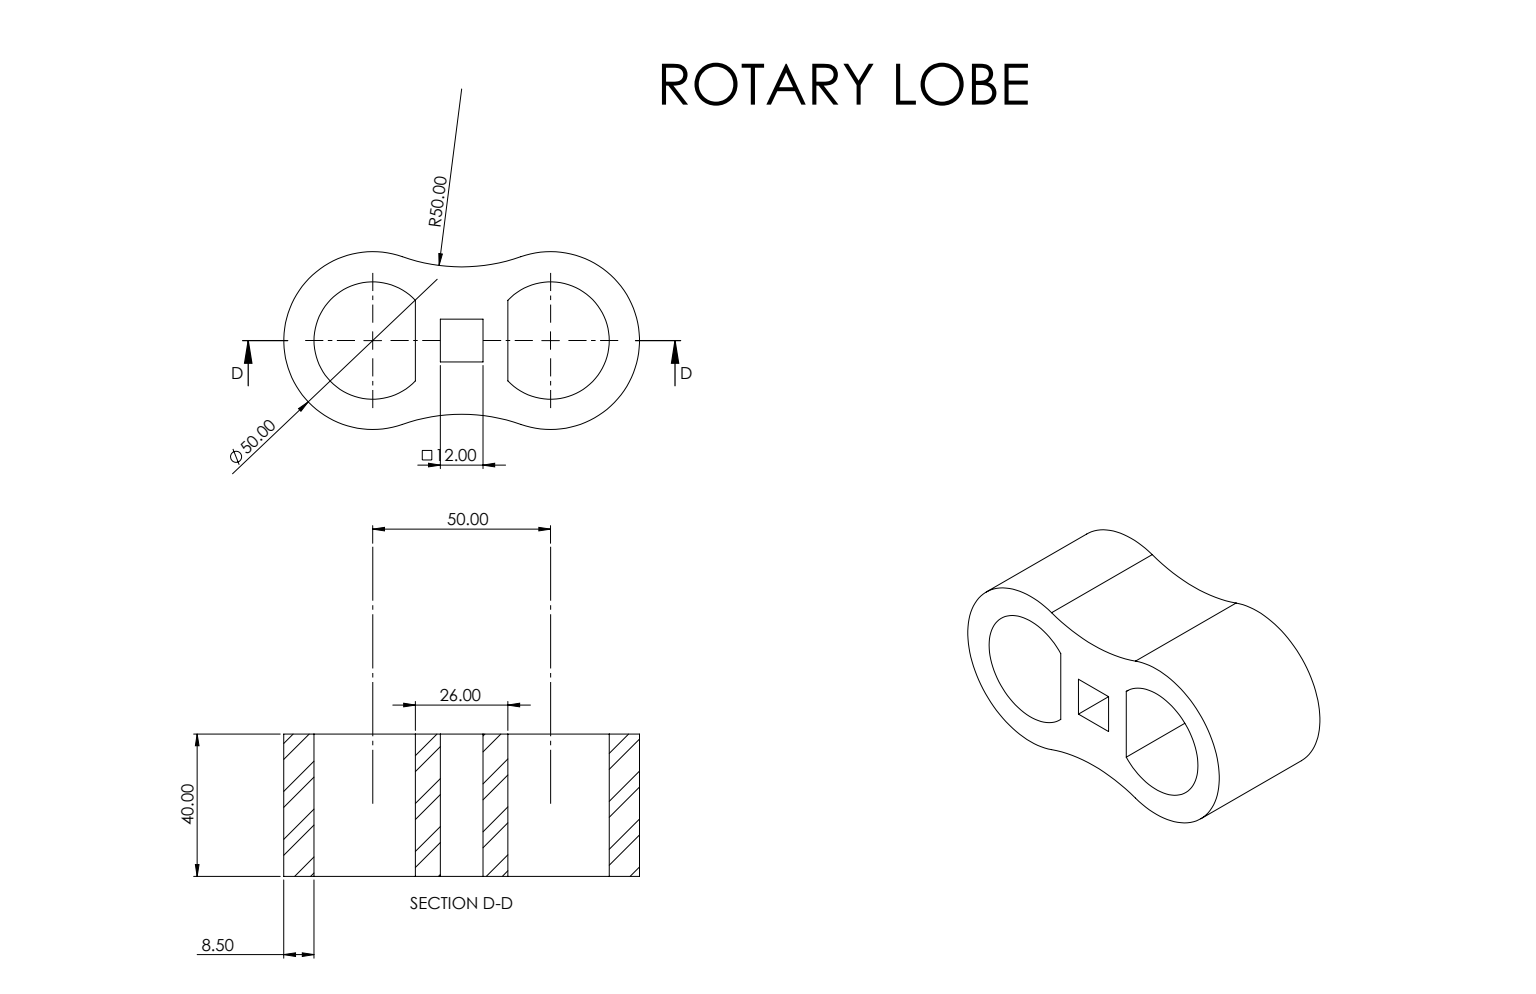
ISO-10303-21;
HEADER;
FILE_DESCRIPTION (('STEP AP214'),
    '1' );
FILE_NAME ('ROTARY LOBE.step',
    '2026-10-24T00:51:42',
    ( '' ),
    ( '' ),
    'SwSTEP 2.0',
    'SolidWorks 2025',
    '' );
FILE_SCHEMA (( 'AUTOMOTIVE_DESIGN' ));
ENDSEC;

DATA;
#53=DIRECTION ( 'NONE',  ( 0.000000000000000000, 0.000000000000000000, 1.000000000000000000 ) ) ;
#96=DIRECTION ( 'NONE',  ( -3.063596499322170048E-16, -0.000000000000000000, -1.000000000000000000 ) ) ;
#131=VERTEX_POINT ( 'NONE', #4797 ) ;
#159=VERTEX_POINT ( 'NONE', #1574 ) ;
#190=EDGE_CURVE ( 'NONE', #16687, #2945, #6029, .T. ) ;
#243=LINE ( 'NONE', #20894, #20346 ) ;
#257=ORIENTED_EDGE ( 'NONE', *, *, #16349, .T. ) ;
#306=PRODUCT_DEFINITION ( 'UNKNOWN', '', #18641, #21271 ) ;
#321=LINE ( 'NONE', #15778, #8511 ) ;
#407=VERTEX_POINT ( 'NONE', #7982 ) ;
#426=DIRECTION ( 'NONE',  ( -3.063596499322173499E-16, 0.000000000000000000, 1.000000000000000000 ) ) ;
#455=CYLINDRICAL_SURFACE ( 'NONE', #13115, 25.00000000000000000 ) ;
#462=DIRECTION ( 'NONE',  ( 0.000000000000000000, -0.000000000000000000, 1.000000000000000000 ) ) ;
#476=EDGE_CURVE ( 'NONE', #15630, #19286, #14390, .T. ) ;
#491=ORIENTED_EDGE ( 'NONE', *, *, #16782, .F. ) ;
#553=AXIS2_PLACEMENT_3D ( 'NONE', #10105, #20446, #6915 ) ;
#568=ORIENTED_EDGE ( 'NONE', *, *, #3531, .T. ) ;
#602=CARTESIAN_POINT ( 'NONE',  ( 25.00000000000000000, -20.00000000000000000, 6.487780019669002523E-15 ) ) ;
#631=DIRECTION ( 'NONE',  ( -0.000000000000000000, -1.000000000000000000, -0.000000000000000000 ) ) ;
#704=CARTESIAN_POINT ( 'NONE',  ( -5.999999999999998224, -20.00000000000000000, 5.999999999999999112 ) ) ;
#705=FACE_OUTER_BOUND ( 'NONE', #13898, .T. ) ;
#723=DIRECTION ( 'NONE',  ( 0.000000000000000000, 1.000000000000000000, -0.000000000000000000 ) ) ;
#779=CARTESIAN_POINT ( 'NONE',  ( -25.00000000000000000, -20.00000000000000000, 6.487780019669002523E-15 ) ) ;
#788=CARTESIAN_POINT ( 'NONE',  ( 12.99999999999999467, -20.00000000000000000, 11.32475165290614605 ) ) ;
#814=AXIS2_PLACEMENT_3D ( 'NONE', #20289, #11347, #21901 ) ;
#880=DIRECTION ( 'NONE',  ( 1.000000000000000000, 0.000000000000000000, 0.000000000000000000 ) ) ;
#893=EDGE_CURVE ( 'NONE', #11565, #12042, #19927, .T. ) ;
#919=AXIS2_PLACEMENT_3D ( 'NONE', #9251, #2386, #7658 ) ;
#965=ORIENTED_EDGE ( 'NONE', *, *, #15758, .T. ) ;
#974=VECTOR ( 'NONE', #96, 1000.000000000000000 ) ;
#989=CYLINDRICAL_SURFACE ( 'NONE', #17809, 16.49999999999998579 ) ;
#1008=DIRECTION ( 'NONE',  ( 0.000000000000000000, 1.000000000000000000, 0.000000000000000000 ) ) ;
#1069=EDGE_CURVE ( 'NONE', #407, #1418, #13674, .T. ) ;
#1071=FACE_OUTER_BOUND ( 'NONE', #3229, .T. ) ;
#1125=DIRECTION ( 'NONE',  ( 0.000000000000000000, 0.000000000000000000, -1.000000000000000000 ) ) ;
#1146=LINE ( 'NONE', #22009, #3920 ) ;
#1355=VECTOR ( 'NONE', #1852, 1000.000000000000000 ) ;
#1369=DIRECTION ( 'NONE',  ( -0.000000000000000000, -1.000000000000000000, -0.000000000000000000 ) ) ;
#1382=EDGE_CURVE ( 'NONE', #2473, #2421, #19105, .T. ) ;
#1401=CARTESIAN_POINT ( 'NONE',  ( -5.999999999999998224, 20.00000000000000000, 5.999999999999999112 ) ) ;
#1413=AXIS2_PLACEMENT_3D ( 'NONE', #7347, #12483, #462 ) ;
#1418=VERTEX_POINT ( 'NONE', #6415 ) ;
#1426=DIRECTION ( 'NONE',  ( 0.000000000000000000, 1.000000000000000000, 0.000000000000000000 ) ) ;
#1447=ORIENTED_EDGE ( 'NONE', *, *, #21089, .F. ) ;
#1523=DIRECTION ( 'NONE',  ( 0.000000000000000000, 0.000000000000000000, -1.000000000000000000 ) ) ;
#1574=CARTESIAN_POINT ( 'NONE',  ( -6.000000000000000000, -20.00000000000000000, -5.999999999999999112 ) ) ;
#1589=DIRECTION ( 'NONE',  ( 3.063596499322170048E-16, 0.000000000000000000, 1.000000000000000000 ) ) ;
#1621=DIRECTION ( 'NONE',  ( -0.000000000000000000, -1.000000000000000000, -0.000000000000000000 ) ) ;
#1648=CARTESIAN_POINT ( 'NONE',  ( 0.000000000000000000, 0.000000000000000000, 0.000000000000000000 ) ) ;
#1741=DIRECTION ( 'NONE',  ( 0.000000000000000000, 1.000000000000000000, 0.000000000000000000 ) ) ;
#1761=ORIENTED_EDGE ( 'NONE', *, *, #17671, .T. ) ;
#1773=DIRECTION ( 'NONE',  ( 0.000000000000000000, 0.000000000000000000, 1.000000000000000000 ) ) ;
#1790=AXIS2_PLACEMENT_3D ( 'NONE', #4562, #17989, #11540 ) ;
#1820=ORIENTED_EDGE ( 'NONE', *, *, #13645, .F. ) ;
#1849=CARTESIAN_POINT ( 'NONE',  ( -25.00000000000000000, 20.00000000000000000, 6.487780019669002523E-15 ) ) ;
#1852=DIRECTION ( 'NONE',  ( 1.445602896647339410E-16, 0.000000000000000000, 1.000000000000000000 ) ) ;
#1858=LINE ( 'NONE', #7117, #6849 ) ;
#1899=EDGE_LOOP ( 'NONE', ( #18124, #14504, #19988, #8484 ) ) ;
#1909=CARTESIAN_POINT ( 'NONE',  ( -25.00000000000000000, -20.00000000000000000, 6.487780019669002523E-15 ) ) ;
#1911=CARTESIAN_POINT ( 'NONE',  ( -16.66666666666665719, 20.00000000000000000, 23.57022603955159923 ) ) ;
#1936=ORIENTED_EDGE ( 'NONE', *, *, #18548, .F. ) ;
#2015=VERTEX_POINT ( 'NONE', #14566 ) ;
#2019=DIRECTION ( 'NONE',  ( 0.000000000000000000, 0.000000000000000000, 1.000000000000000000 ) ) ;
#2030=VERTEX_POINT ( 'NONE', #21576 ) ;
#2094=DIRECTION ( 'NONE',  ( 0.000000000000000000, 1.000000000000000000, -0.000000000000000000 ) ) ;
#2095=EDGE_LOOP ( 'NONE', ( #17339, #14563, #19602, #12820, #491, #11785, #13566, #22488, #22666 ) ) ;
#2119=ORIENTED_EDGE ( 'NONE', *, *, #11671, .T. ) ;
#2141=DIRECTION ( 'NONE',  ( -0.000000000000000000, -1.000000000000000000, -0.000000000000000000 ) ) ;
#2174=EDGE_LOOP ( 'NONE', ( #6678, #9947, #19944, #8878 ) ) ;
#2198=CIRCLE ( 'NONE', #18295, 25.00000000000000711 ) ;
#2229=AXIS2_PLACEMENT_3D ( 'NONE', #3378, #1426, #5315 ) ;
#2248=CARTESIAN_POINT ( 'NONE',  ( 25.00000000000000000, 20.00000000000000000, 6.487780019669002523E-15 ) ) ;
#2250=DIRECTION ( 'NONE',  ( 0.000000000000000000, 0.000000000000000000, 1.000000000000000000 ) ) ;
#2259=CARTESIAN_POINT ( 'NONE',  ( -5.999999999999998224, -20.00000000000000000, 5.999999999999999112 ) ) ;
#2279=CARTESIAN_POINT ( 'NONE',  ( 13.00000000000000178, 20.00000000000000000, -11.32475165290605901 ) ) ;
#2306=DIRECTION ( 'NONE',  ( -1.000000000000000000, 0.000000000000000000, 1.445602896647339410E-16 ) ) ;
#2312=ORIENTED_EDGE ( 'NONE', *, *, #5126, .F. ) ;
#2339=AXIS2_PLACEMENT_3D ( 'NONE', #13019, #1008, #21638 ) ;
#2378=LINE ( 'NONE', #18404, #11244 ) ;
#2386=DIRECTION ( 'NONE',  ( 0.000000000000000000, 1.000000000000000000, -0.000000000000000000 ) ) ;
#2421=VERTEX_POINT ( 'NONE', #8784 ) ;
#2433=EDGE_CURVE ( 'NONE', #17903, #10299, #3295, .T. ) ;
#2468=VECTOR ( 'NONE', #5542, 1000.000000000000000 ) ;
#2473=VERTEX_POINT ( 'NONE', #17595 ) ;
#2693=VERTEX_POINT ( 'NONE', #15154 ) ;
#2698=CARTESIAN_POINT ( 'NONE',  ( 12.99999999999999467, 20.00000000000000000, 11.32475165290614960 ) ) ;
#2712=DIRECTION ( 'NONE',  ( 0.000000000000000000, 1.000000000000000000, -0.000000000000000000 ) ) ;
#2728=FACE_OUTER_BOUND ( 'NONE', #6014, .T. ) ;
#2780=DIRECTION ( 'NONE',  ( -1.445602896647339410E-16, 0.000000000000000000, -1.000000000000000000 ) ) ;
#2792=LINE ( 'NONE', #4512, #19358 ) ;
#2818=DIRECTION ( 'NONE',  ( 0.000000000000000000, 1.000000000000000000, -0.000000000000000000 ) ) ;
#2827=ORIENTED_EDGE ( 'NONE', *, *, #14634, .T. ) ;
#2839=EDGE_CURVE ( 'NONE', #12042, #15630, #21166, .T. ) ;
#2900=( GEOMETRIC_REPRESENTATION_CONTEXT ( 3 ) GLOBAL_UNCERTAINTY_ASSIGNED_CONTEXT ( ( #11243 ) ) GLOBAL_UNIT_ASSIGNED_CONTEXT ( ( #17257, #8792, #12436 ) ) REPRESENTATION_CONTEXT ( 'NONE', 'WORKASPACE' ) );
#2913=DIRECTION ( 'NONE',  ( -0.000000000000000000, -1.000000000000000000, -0.000000000000000000 ) ) ;
#2945=VERTEX_POINT ( 'NONE', #19754 ) ;
#2970=CARTESIAN_POINT ( 'NONE',  ( -25.00000000000000000, 20.00000000000000000, -25.00000000000000000 ) ) ;
#2974=ORIENTED_EDGE ( 'NONE', *, *, #2433, .T. ) ;
#3037=ORIENTED_EDGE ( 'NONE', *, *, #16349, .F. ) ;
#3046=CARTESIAN_POINT ( 'NONE',  ( 16.66666666666669272, 20.00000000000000000, -23.57022603955159212 ) ) ;
#3095=LINE ( 'NONE', #14993, #11566 ) ;
#3102=AXIS2_PLACEMENT_3D ( 'NONE', #20493, #18423, #16830 ) ;
#3121=PLANE ( 'NONE',  #6042 ) ;
#3124=DIRECTION ( 'NONE',  ( 0.000000000000000000, 0.000000000000000000, 1.000000000000000000 ) ) ;
#3169=ORIENTED_EDGE ( 'NONE', *, *, #9920, .T. ) ;
#3200=ORIENTED_EDGE ( 'NONE', *, *, #6746, .F. ) ;
#3216=DIRECTION ( 'NONE',  ( 0.000000000000000000, 1.000000000000000000, 0.000000000000000000 ) ) ;
#3229=EDGE_LOOP ( 'NONE', ( #3200, #2312, #7838, #18951 ) ) ;
#3261=ORIENTED_EDGE ( 'NONE', *, *, #21083, .T. ) ;
#3262=AXIS2_PLACEMENT_3D ( 'NONE', #1849, #1621, #6664 ) ;
#3272=ADVANCED_FACE ( 'NONE', ( #15357 ), #10536, .T. ) ;
#3283=CIRCLE ( 'NONE', #18637, 25.00000000000000000 ) ;
#3295=LINE ( 'NONE', #19440, #19357 ) ;
#3327=LINE ( 'NONE', #6750, #20585 ) ;
#3378=CARTESIAN_POINT ( 'NONE',  ( -25.00000000000000000, 20.00000000000000000, 6.487780019669002523E-15 ) ) ;
#3430=SHAPE_REPRESENTATION ( 'ROTARY LOBE', ( #18273 ), #17150 ) ;
#3442=LINE ( 'NONE', #5489, #974 ) ;
#3484=CLOSED_SHELL ( 'NONE', ( #18863, #5857, #19734, #13310, #7530, #19685, #18289, #19085, #21947, #10343, #10632, #16278, #3272, #14244, #20666, #16635, #19070, #18858, #14622, #18536, #12603, #19793, #5819 ) ) ;
#3490=CARTESIAN_POINT ( 'NONE',  ( -12.99999999999999289, 20.00000000000000000, 11.32475165290611940 ) ) ;
#3521=VECTOR ( 'NONE', #15900, 1000.000000000000000 ) ;
#3531=EDGE_CURVE ( 'NONE', #2015, #20188, #12586, .T. ) ;
#3564=ORIENTED_EDGE ( 'NONE', *, *, #7437, .T. ) ;
#3585=ORIENTED_EDGE ( 'NONE', *, *, #21827, .F. ) ;
#3668=VECTOR ( 'NONE', #2141, 1000.000000000000000 ) ;
#3749=DIRECTION ( 'NONE',  ( 0.000000000000000000, 1.000000000000000000, 0.000000000000000000 ) ) ;
#3763=EDGE_CURVE ( 'NONE', #2693, #10299, #3327, .T. ) ;
#3765=CIRCLE ( 'NONE', #18773, 25.00000000000000000 ) ;
#3789=DIRECTION ( 'NONE',  ( 0.000000000000000000, 1.000000000000000000, 0.000000000000000000 ) ) ;
#3835=CARTESIAN_POINT ( 'NONE',  ( -16.66666666666665719, -20.00000000000000000, 23.57022603955159923 ) ) ;
#3837=AXIS2_PLACEMENT_3D ( 'NONE', #8979, #3838, #7382 ) ;
#3838=DIRECTION ( 'NONE',  ( 0.000000000000000000, 1.000000000000000000, 0.000000000000000000 ) ) ;
#3856=ORIENTED_EDGE ( 'NONE', *, *, #14469, .F. ) ;
#3860=EDGE_CURVE ( 'NONE', #17205, #20094, #321, .T. ) ;
#3864=CARTESIAN_POINT ( 'NONE',  ( -24.99999999999999645, 20.00000000000000000, 25.00000000000001421 ) ) ;
#3910=CARTESIAN_POINT ( 'NONE',  ( 5.999999999999998224, 20.00000000000000000, -5.999999999999999112 ) ) ;
#3920=VECTOR ( 'NONE', #22353, 1000.000000000000000 ) ;
#3955=VECTOR ( 'NONE', #12617, 1000.000000000000000 ) ;
#4012=DIRECTION ( 'NONE',  ( -0.000000000000000000, -1.000000000000000000, -0.000000000000000000 ) ) ;
#4017=AXIS2_PLACEMENT_3D ( 'NONE', #9577, #2712, #20128 ) ;
#4039=CARTESIAN_POINT ( 'NONE',  ( 25.00000000000000000, 20.00000000000000000, 6.487780019669002523E-15 ) ) ;
#4121=FACE_OUTER_BOUND ( 'NONE', #5496, .T. ) ;
#4164=CARTESIAN_POINT ( 'NONE',  ( -25.00000000000000000, 20.00000000000000000, -16.49999999999998934 ) ) ;
#4227=VECTOR ( 'NONE', #12091, 1000.000000000000000 ) ;
#4269=ORIENTED_EDGE ( 'NONE', *, *, #16752, .T. ) ;
#4276=DIRECTION ( 'NONE',  ( -0.000000000000000000, -1.000000000000000000, 0.000000000000000000 ) ) ;
#4325=AXIS2_PLACEMENT_3D ( 'NONE', #15578, #3789, #22601 ) ;
#4396=CARTESIAN_POINT ( 'NONE',  ( -25.00000000000000000, 20.00000000000000000, 6.487780019669002523E-15 ) ) ;
#4449=DIRECTION ( 'NONE',  ( 0.000000000000000000, 1.000000000000000000, 0.000000000000000000 ) ) ;
#4454=ORIENTED_EDGE ( 'NONE', *, *, #893, .T. ) ;
#4512=CARTESIAN_POINT ( 'NONE',  ( -16.66666666666665719, 20.00000000000000000, 23.57022603955159923 ) ) ;
#4516=EDGE_CURVE ( 'NONE', #5200, #16687, #22138, .T. ) ;
#4517=ORIENTED_EDGE ( 'NONE', *, *, #11352, .F. ) ;
#4562=CARTESIAN_POINT ( 'NONE',  ( -25.00000000000000000, 20.00000000000000000, 6.487780019669002523E-15 ) ) ;
#4571=DIRECTION ( 'NONE',  ( -0.000000000000000000, -1.000000000000000000, -0.000000000000000000 ) ) ;
#4602=CARTESIAN_POINT ( 'NONE',  ( 1.734723475976807094E-14, -20.00000000000000000, 70.71067811865476926 ) ) ;
#4624=DIRECTION ( 'NONE',  ( -0.000000000000000000, -1.000000000000000000, -0.000000000000000000 ) ) ;
#4657=CARTESIAN_POINT ( 'NONE',  ( 5.999999999999998224, -20.00000000000000000, -5.999999999999999112 ) ) ;
#4662=CARTESIAN_POINT ( 'NONE',  ( 1.734723475976807094E-14, -20.00000000000000000, 70.71067811865476926 ) ) ;
#4702=VECTOR ( 'NONE', #426, 1000.000000000000000 ) ;
#4754=CARTESIAN_POINT ( 'NONE',  ( -6.000000000000000000, 20.00000000000000000, -5.999999999999999112 ) ) ;
#4770=AXIS2_PLACEMENT_3D ( 'NONE', #15418, #4571, #1125 ) ;
#4796=ORIENTED_EDGE ( 'NONE', *, *, #20868, .F. ) ;
#4797=CARTESIAN_POINT ( 'NONE',  ( 25.00000000000000000, -20.00000000000000000, -24.99999999999999289 ) ) ;
#4835=CARTESIAN_POINT ( 'NONE',  ( -25.00000000000000000, 20.00000000000000000, 6.487780019669002523E-15 ) ) ;
#4867=LINE ( 'NONE', #13888, #5896 ) ;
#4885=ORIENTED_EDGE ( 'NONE', *, *, #9185, .T. ) ;
#4921=DIRECTION ( 'NONE',  ( -1.000000000000000000, 0.000000000000000000, 3.063596499322170048E-16 ) ) ;
#4932=CARTESIAN_POINT ( 'NONE',  ( -24.99999999999999645, 20.00000000000000000, 16.50000000000000355 ) ) ;
#4958=CARTESIAN_POINT ( 'NONE',  ( 25.00000000000000000, 20.00000000000000000, 6.487780019669002523E-15 ) ) ;
#4980=CARTESIAN_POINT ( 'NONE',  ( -25.00000000000000000, -20.00000000000000000, 6.487780019669002523E-15 ) ) ;
#4983=CIRCLE ( 'NONE', #6815, 16.49999999999999645 ) ;
#5034=LINE ( 'NONE', #6406, #18207 ) ;
#5063=SHAPE_DEFINITION_REPRESENTATION ( #14396, #3430 ) ;
#5089=CARTESIAN_POINT ( 'NONE',  ( -25.00000000000000000, 20.00000000000000000, 6.487780019669002523E-15 ) ) ;
#5126=EDGE_CURVE ( 'NONE', #11767, #20985, #19755, .T. ) ;
#5128=DIRECTION ( 'NONE',  ( -3.063596499322170048E-16, -0.000000000000000000, -1.000000000000000000 ) ) ;
#5158=FACE_OUTER_BOUND ( 'NONE', #5317, .T. ) ;
#5200=VERTEX_POINT ( 'NONE', #4164 ) ;
#5251=CIRCLE ( 'NONE', #3837, 25.00000000000000000 ) ;
#5272=LINE ( 'NONE', #11789, #21724 ) ;
#5281=AXIS2_PLACEMENT_3D ( 'NONE', #7089, #3216, #15441 ) ;
#5315=DIRECTION ( 'NONE',  ( 0.000000000000000000, 0.000000000000000000, 1.000000000000000000 ) ) ;
#5317=EDGE_LOOP ( 'NONE', ( #10062, #14422, #7754, #15956 ) ) ;
#5371=CARTESIAN_POINT ( 'NONE',  ( -25.00000000000000000, 20.00000000000000000, 6.487780019669002523E-15 ) ) ;
#5418=ORIENTED_EDGE ( 'NONE', *, *, #3860, .F. ) ;
#5489=CARTESIAN_POINT ( 'NONE',  ( -13.00000000000000178, 20.00000000000000000, -11.32475165290611407 ) ) ;
#5492=CARTESIAN_POINT ( 'NONE',  ( -5.999999999999998224, 20.00000000000000000, 5.999999999999999112 ) ) ;
#5496=EDGE_LOOP ( 'NONE', ( #9868, #6218, #10357, #19825 ) ) ;
#5516=DIRECTION ( 'NONE',  ( -0.000000000000000000, -1.000000000000000000, -0.000000000000000000 ) ) ;
#5542=DIRECTION ( 'NONE',  ( -0.000000000000000000, -1.000000000000000000, -0.000000000000000000 ) ) ;
#5613=DIRECTION ( 'NONE',  ( -0.000000000000000000, -1.000000000000000000, -0.000000000000000000 ) ) ;
#5628=VECTOR ( 'NONE', #880, 1000.000000000000000 ) ;
#5630=VERTEX_POINT ( 'NONE', #11344 ) ;
#5653=CARTESIAN_POINT ( 'NONE',  ( 25.00000000000000355, 20.00000000000000000, 16.49999999999999289 ) ) ;
#5715=ORIENTED_EDGE ( 'NONE', *, *, #17671, .F. ) ;
#5755=( NAMED_UNIT ( * ) SI_UNIT ( $, .STERADIAN. ) SOLID_ANGLE_UNIT ( ) );
#5768=DIRECTION ( 'NONE',  ( 0.000000000000000000, 0.000000000000000000, 1.000000000000000000 ) ) ;
#5819=ADVANCED_FACE ( 'NONE', ( #5158 ), #6983, .T. ) ;
#5829=PRODUCT ( 'ROTARY LOBE', 'ROTARY LOBE', '', ( #10300 ) ) ;
#5840=DIRECTION ( 'NONE',  ( 1.000000000000000000, -0.000000000000000000, 3.063596499322173499E-16 ) ) ;
#5857=ADVANCED_FACE ( 'NONE', ( #12023 ), #15673, .F. ) ;
#5892=DIRECTION ( 'NONE',  ( 1.000000000000000000, 0.000000000000000000, -0.000000000000000000 ) ) ;
#5896=VECTOR ( 'NONE', #19298, 1000.000000000000000 ) ;
#5949=EDGE_CURVE ( 'NONE', #11275, #11481, #9145, .T. ) ;
#5975=ORIENTED_EDGE ( 'NONE', *, *, #12491, .F. ) ;
#5999=LINE ( 'NONE', #7490, #7179 ) ;
#6014=EDGE_LOOP ( 'NONE', ( #13694, #2827, #8705, #18362 ) ) ;
#6028=EDGE_CURVE ( 'NONE', #2421, #11565, #13451, .T. ) ;
#6029=CIRCLE ( 'NONE', #18836, 16.49999999999999645 ) ;
#6030=DIRECTION ( 'NONE',  ( 0.000000000000000000, 1.000000000000000000, 0.000000000000000000 ) ) ;
#6041=DIRECTION ( 'NONE',  ( 1.445602896647339410E-16, 0.000000000000000000, 1.000000000000000000 ) ) ;
#6042=AXIS2_PLACEMENT_3D ( 'NONE', #1401, #8059, #15362 ) ;
#6048=LINE ( 'NONE', #13015, #15559 ) ;
#6117=DIRECTION ( 'NONE',  ( -0.000000000000000000, -1.000000000000000000, -0.000000000000000000 ) ) ;
#6161=LINE ( 'NONE', #2259, #5628 ) ;
#6218=ORIENTED_EDGE ( 'NONE', *, *, #9082, .F. ) ;
#6330=LINE ( 'NONE', #13289, #10426 ) ;
#6337=EDGE_CURVE ( 'NONE', #17762, #15630, #2792, .T. ) ;
#6406=CARTESIAN_POINT ( 'NONE',  ( -25.00000000000000000, 20.00000000000000000, -25.00000000000000000 ) ) ;
#6415=CARTESIAN_POINT ( 'NONE',  ( 13.00000000000000178, 20.00000000000000000, -11.32475165290605723 ) ) ;
#6436=CARTESIAN_POINT ( 'NONE',  ( -25.00000000000000000, 20.00000000000000000, -16.49999999999998934 ) ) ;
#6458=FACE_OUTER_BOUND ( 'NONE', #7366, .T. ) ;
#6459=FACE_OUTER_BOUND ( 'NONE', #9454, .T. ) ;
#6555=FACE_OUTER_BOUND ( 'NONE', #18849, .T. ) ;
#6598=DIRECTION ( 'NONE',  ( -0.000000000000000000, -1.000000000000000000, 0.000000000000000000 ) ) ;
#6649=DIRECTION ( 'NONE',  ( -0.000000000000000000, -1.000000000000000000, -0.000000000000000000 ) ) ;
#6664=DIRECTION ( 'NONE',  ( 0.000000000000000000, 0.000000000000000000, -1.000000000000000000 ) ) ;
#6675=CYLINDRICAL_SURFACE ( 'NONE', #20729, 25.00000000000000000 ) ;
#6678=ORIENTED_EDGE ( 'NONE', *, *, #15968, .F. ) ;
#6700=EDGE_LOOP ( 'NONE', ( #9292, #1761, #17911, #7155 ) ) ;
#6720=DIRECTION ( 'NONE',  ( -0.000000000000000000, -1.000000000000000000, -0.000000000000000000 ) ) ;
#6746=EDGE_CURVE ( 'NONE', #20985, #9978, #6161, .T. ) ;
#6750=CARTESIAN_POINT ( 'NONE',  ( -13.00000000000000178, 20.00000000000000000, -11.32475165290611407 ) ) ;
#6763=DIRECTION ( 'NONE',  ( 0.000000000000000000, 0.000000000000000000, -1.000000000000000000 ) ) ;
#6815=AXIS2_PLACEMENT_3D ( 'NONE', #4396, #16528, #5768 ) ;
#6849=VECTOR ( 'NONE', #14663, 1000.000000000000000 ) ;
#6866=CIRCLE ( 'NONE', #4325, 25.00000000000000000 ) ;
#6903=CARTESIAN_POINT ( 'NONE',  ( -25.00000000000000000, -20.00000000000000000, 6.487780019669002523E-15 ) ) ;
#6915=DIRECTION ( 'NONE',  ( 0.000000000000000000, 0.000000000000000000, -1.000000000000000000 ) ) ;
#6983=PLANE ( 'NONE',  #11266 ) ;
#6988=FACE_BOUND ( 'NONE', #8101, .T. ) ;
#6994=DIRECTION ( 'NONE',  ( 0.000000000000000000, 0.000000000000000000, 1.000000000000000000 ) ) ;
#7089=CARTESIAN_POINT ( 'NONE',  ( 12.50000000000000888, -20.00000000000000000, -35.35533905932738463 ) ) ;
#7117=CARTESIAN_POINT ( 'NONE',  ( -24.99999999999999645, 20.00000000000000000, 16.50000000000000355 ) ) ;
#7155=ORIENTED_EDGE ( 'NONE', *, *, #5949, .T. ) ;
#7176=AXIS2_PLACEMENT_3D ( 'NONE', #11793, #8145, #14999 ) ;
#7179=VECTOR ( 'NONE', #6117, 1000.000000000000000 ) ;
#7291=VERTEX_POINT ( 'NONE', #2698 ) ;
#7324=VERTEX_POINT ( 'NONE', #14931 ) ;
#7347=CARTESIAN_POINT ( 'NONE',  ( 12.50000000000000888, 20.00000000000000000, -35.35533905932738463 ) ) ;
#7360=( LENGTH_UNIT ( ) NAMED_UNIT ( * ) SI_UNIT ( .MILLI., .METRE. ) );
#7366=EDGE_LOOP ( 'NONE', ( #1936, #14220, #9943, #22495 ) ) ;
#7369=ORIENTED_EDGE ( 'NONE', *, *, #18515, .F. ) ;
#7382=DIRECTION ( 'NONE',  ( 0.000000000000000000, 0.000000000000000000, 1.000000000000000000 ) ) ;
#7405=CYLINDRICAL_SURFACE ( 'NONE', #10592, 16.49999999999998579 ) ;
#7412=ORIENTED_EDGE ( 'NONE', *, *, #1069, .T. ) ;
#7437=EDGE_CURVE ( 'NONE', #16688, #12891, #8914, .T. ) ;
#7490=CARTESIAN_POINT ( 'NONE',  ( -12.99999999999999467, 20.00000000000000000, 11.32475165290612296 ) ) ;
#7530=ADVANCED_FACE ( 'NONE', ( #18165 ), #11164, .T. ) ;
#7549=EDGE_LOOP ( 'NONE', ( #3169, #12624, #4885, #2974 ) ) ;
#7601=AXIS2_PLACEMENT_3D ( 'NONE', #18464, #10083, #2780 ) ;
#7608=DIRECTION ( 'NONE',  ( 0.000000000000000000, 0.000000000000000000, 1.000000000000000000 ) ) ;
#7658=DIRECTION ( 'NONE',  ( 0.000000000000000000, 0.000000000000000000, -1.000000000000000000 ) ) ;
#7671=ORIENTED_EDGE ( 'NONE', *, *, #18661, .F. ) ;
#7687=FACE_BOUND ( 'NONE', #1899, .T. ) ;
#7698=ORIENTED_EDGE ( 'NONE', *, *, #7997, .T. ) ;
#7749=EDGE_CURVE ( 'NONE', #16771, #7803, #12104, .T. ) ;
#7754=ORIENTED_EDGE ( 'NONE', *, *, #15877, .T. ) ;
#7775=EDGE_CURVE ( 'NONE', #2030, #9978, #4867, .T. ) ;
#7803=VERTEX_POINT ( 'NONE', #3490 ) ;
#7838=ORIENTED_EDGE ( 'NONE', *, *, #13992, .T. ) ;
#7872=AXIS2_PLACEMENT_3D ( 'NONE', #4662, #6598, #13562 ) ;
#7938=ORIENTED_EDGE ( 'NONE', *, *, #476, .T. ) ;
#7953=EDGE_LOOP ( 'NONE', ( #1447, #12865, #17410, #2119 ) ) ;
#7982=CARTESIAN_POINT ( 'NONE',  ( 25.00000000000000000, 20.00000000000000000, -16.49999999999997868 ) ) ;
#7985=ORIENTED_EDGE ( 'NONE', *, *, #18946, .T. ) ;
#7990=CIRCLE ( 'NONE', #18236, 16.49999999999999645 ) ;
#7997=EDGE_CURVE ( 'NONE', #17762, #10374, #22371, .T. ) ;
#8000=FACE_OUTER_BOUND ( 'NONE', #21573, .T. ) ;
#8059=DIRECTION ( 'NONE',  ( 0.000000000000000000, 0.000000000000000000, -1.000000000000000000 ) ) ;
#8101=EDGE_LOOP ( 'NONE', ( #965, #15077, #19109, #13023 ) ) ;
#8105=FACE_OUTER_BOUND ( 'NONE', #10982, .T. ) ;
#8145=DIRECTION ( 'NONE',  ( 0.000000000000000000, 1.000000000000000000, 0.000000000000000000 ) ) ;
#8174=DIRECTION ( 'NONE',  ( -0.000000000000000000, -1.000000000000000000, -0.000000000000000000 ) ) ;
#8175=DIRECTION ( 'NONE',  ( 0.000000000000000000, 1.000000000000000000, 0.000000000000000000 ) ) ;
#8222=AXIS2_PLACEMENT_3D ( 'NONE', #9939, #13699, #17038 ) ;
#8233=EDGE_LOOP ( 'NONE', ( #17203, #16857, #11709, #19544 ) ) ;
#8344=AXIS2_PLACEMENT_3D ( 'NONE', #20252, #6720, #11536 ) ;
#8364=VERTEX_POINT ( 'NONE', #14301 ) ;
#8369=ORIENTED_EDGE ( 'NONE', *, *, #17783, .T. ) ;
#8371=CARTESIAN_POINT ( 'NONE',  ( 1.734723475976807094E-14, 20.00000000000000000, -70.71067811865476926 ) ) ;
#8382=CYLINDRICAL_SURFACE ( 'NONE', #17110, 16.49999999999999645 ) ;
#8384=VERTEX_POINT ( 'NONE', #10994 ) ;
#8396=FACE_OUTER_BOUND ( 'NONE', #7953, .T. ) ;
#8484=ORIENTED_EDGE ( 'NONE', *, *, #17041, .F. ) ;
#8507=CYLINDRICAL_SURFACE ( 'NONE', #553, 50.00000000000001421 ) ;
#8511=VECTOR ( 'NONE', #21521, 1000.000000000000000 ) ;
#8522=ORIENTED_EDGE ( 'NONE', *, *, #11352, .T. ) ;
#8594=ORIENTED_EDGE ( 'NONE', *, *, #13992, .F. ) ;
#8623=VECTOR ( 'NONE', #10210, 1000.000000000000000 ) ;
#8698=AXIS2_PLACEMENT_3D ( 'NONE', #5371, #21522, #12791 ) ;
#8705=ORIENTED_EDGE ( 'NONE', *, *, #13539, .T. ) ;
#8772=CARTESIAN_POINT ( 'NONE',  ( 25.00000000000000000, -20.00000000000000000, 6.487780019669002523E-15 ) ) ;
#8784=CARTESIAN_POINT ( 'NONE',  ( -16.66666666666666785, -20.00000000000000000, -23.57022603955158502 ) ) ;
#8792=( NAMED_UNIT ( * ) PLANE_ANGLE_UNIT ( ) SI_UNIT ( $, .RADIAN. ) );
#8850=SHAPE_REPRESENTATION_RELATIONSHIP ( 'NONE' , 'NONE' ,  #3430, #14250 ) ;
#8878=ORIENTED_EDGE ( 'NONE', *, *, #13645, .T. ) ;
#8914=CIRCLE ( 'NONE', #2339, 25.00000000000000711 ) ;
#8943=DIRECTION ( 'NONE',  ( 0.000000000000000000, 0.000000000000000000, -1.000000000000000000 ) ) ;
#8973=VERTEX_POINT ( 'NONE', #10790 ) ;
#8979=CARTESIAN_POINT ( 'NONE',  ( 25.00000000000000000, 20.00000000000000000, 6.487780019669002523E-15 ) ) ;
#8988=VERTEX_POINT ( 'NONE', #17912 ) ;
#9082=EDGE_CURVE ( 'NONE', #1418, #11275, #11600, .T. ) ;
#9128=DIRECTION ( 'NONE',  ( 0.000000000000000000, 0.000000000000000000, -1.000000000000000000 ) ) ;
#9145=LINE ( 'NONE', #16116, #4702 ) ;
#9185=EDGE_CURVE ( 'NONE', #2945, #17903, #20404, .T. ) ;
#9213=EDGE_CURVE ( 'NONE', #159, #20985, #10089, .T. ) ;
#9251=CARTESIAN_POINT ( 'NONE',  ( 25.00000000000000000, -20.00000000000000000, 6.487780019669002523E-15 ) ) ;
#9292=ORIENTED_EDGE ( 'NONE', *, *, #14469, .T. ) ;
#9357=CARTESIAN_POINT ( 'NONE',  ( 25.00000000000000000, 20.00000000000000000, 6.487780019669002523E-15 ) ) ;
#9360=DIRECTION ( 'NONE',  ( -0.000000000000000000, -1.000000000000000000, -0.000000000000000000 ) ) ;
#9368=ORIENTED_EDGE ( 'NONE', *, *, #16106, .F. ) ;
#9437=ORIENTED_EDGE ( 'NONE', *, *, #4516, .F. ) ;
#9454=EDGE_LOOP ( 'NONE', ( #12266, #22168, #5975, #14521 ) ) ;
#9487=MECHANICAL_DESIGN_GEOMETRIC_PRESENTATION_REPRESENTATION('',(#9844),#2900);
#9577=CARTESIAN_POINT ( 'NONE',  ( 25.00000000000000000, 20.00000000000000000, 6.487780019669002523E-15 ) ) ;
#9761=DIRECTION ( 'NONE',  ( 0.000000000000000000, 0.000000000000000000, -1.000000000000000000 ) ) ;
#9762=DIRECTION ( 'NONE',  ( 0.000000000000000000, 0.000000000000000000, -1.000000000000000000 ) ) ;
#9774=CARTESIAN_POINT ( 'NONE',  ( -25.00000000000000000, -20.00000000000000000, 6.487780019669002523E-15 ) ) ;
#9835=CYLINDRICAL_SURFACE ( 'NONE', #4770, 50.00000000000000000 ) ;
#9844=STYLED_ITEM('',(#22720),#17752);
#9850=ORIENTED_EDGE ( 'NONE', *, *, #9185, .F. ) ;
#9868=ORIENTED_EDGE ( 'NONE', *, *, #5949, .F. ) ;
#9884=DIRECTION ( 'NONE',  ( 0.000000000000000000, 1.000000000000000000, 0.000000000000000000 ) ) ;
#9920=EDGE_CURVE ( 'NONE', #10299, #16687, #7990, .T. ) ;
#9939=CARTESIAN_POINT ( 'NONE',  ( 1.734723475976807094E-14, 20.00000000000000000, 70.71067811865476926 ) ) ;
#9943=ORIENTED_EDGE ( 'NONE', *, *, #2839, .T. ) ;
#9947=ORIENTED_EDGE ( 'NONE', *, *, #3531, .F. ) ;
#9978=VERTEX_POINT ( 'NONE', #14374 ) ;
#9987=DIRECTION ( 'NONE',  ( -0.000000000000000000, -1.000000000000000000, -0.000000000000000000 ) ) ;
#9989=ORIENTED_EDGE ( 'NONE', *, *, #11233, .T. ) ;
#10062=ORIENTED_EDGE ( 'NONE', *, *, #2433, .F. ) ;
#10083=DIRECTION ( 'NONE',  ( 1.000000000000000000, 0.000000000000000000, -1.445602896647339410E-16 ) ) ;
#10089=LINE ( 'NONE', #22490, #1355 ) ;
#10105=CARTESIAN_POINT ( 'NONE',  ( 1.734723475976807094E-14, 20.00000000000000000, -70.71067811865476926 ) ) ;
#10180=FACE_BOUND ( 'NONE', #6700, .T. ) ;
#10210=DIRECTION ( 'NONE',  ( -0.000000000000000000, -1.000000000000000000, -0.000000000000000000 ) ) ;
#10217=CYLINDRICAL_SURFACE ( 'NONE', #10507, 25.00000000000000711 ) ;
#10219=DIRECTION ( 'NONE',  ( 0.000000000000000000, 0.000000000000000000, 1.000000000000000000 ) ) ;
#10299=VERTEX_POINT ( 'NONE', #17232 ) ;
#10300=PRODUCT_CONTEXT ( 'NONE', #12230, 'mechanical' ) ;
#10343=ADVANCED_FACE ( 'NONE', ( #705, #16150, #21561, #7687 ), #17995, .T. ) ;
#10357=ORIENTED_EDGE ( 'NONE', *, *, #12295, .T. ) ;
#10368=AXIS2_PLACEMENT_3D ( 'NONE', #2279, #5840, #21081 ) ;
#10374=VERTEX_POINT ( 'NONE', #14315 ) ;
#10409=ORIENTED_EDGE ( 'NONE', *, *, #16566, .F. ) ;
#10426=VECTOR ( 'NONE', #4624, 1000.000000000000000 ) ;
#10430=ORIENTED_EDGE ( 'NONE', *, *, #12491, .T. ) ;
#10438=AXIS2_PLACEMENT_3D ( 'NONE', #14556, #2306, #14776 ) ;
#10507=AXIS2_PLACEMENT_3D ( 'NONE', #15372, #8174, #1523 ) ;
#10536=CYLINDRICAL_SURFACE ( 'NONE', #3262, 25.00000000000000711 ) ;
#10577=ORIENTED_EDGE ( 'NONE', *, *, #7437, .F. ) ;
#10592=AXIS2_PLACEMENT_3D ( 'NONE', #9357, #21388, #9128 ) ;
#10632=ADVANCED_FACE ( 'NONE', ( #10180, #17521, #6988, #18908 ), #13944, .F. ) ;
#10721=AXIS2_PLACEMENT_3D ( 'NONE', #8371, #6649, #6994 ) ;
#10725=EDGE_CURVE ( 'NONE', #17205, #8364, #5251, .T. ) ;
#10761=EDGE_LOOP ( 'NONE', ( #11696, #14892, #20306, #5418 ) ) ;
#10774=CIRCLE ( 'NONE', #919, 16.49999999999998579 ) ;
#10790=CARTESIAN_POINT ( 'NONE',  ( 25.00000000000000000, -20.00000000000000000, -16.49999999999997868 ) ) ;
#10819=DIRECTION ( 'NONE',  ( 0.000000000000000000, 0.000000000000000000, -1.000000000000000000 ) ) ;
#10863=PLANE ( 'NONE',  #10368 ) ;
#10961=EDGE_LOOP ( 'NONE', ( #18458, #10577, #12982, #18087 ) ) ;
#10982=EDGE_LOOP ( 'NONE', ( #7369, #3037, #15035, #4454 ) ) ;
#10994=CARTESIAN_POINT ( 'NONE',  ( 25.00000000000000355, -20.00000000000000000, 16.49999999999999289 ) ) ;
#11038=CARTESIAN_POINT ( 'NONE',  ( 16.66666666666669272, 20.00000000000000000, -23.57022603955159212 ) ) ;
#11059=DIRECTION ( 'NONE',  ( 0.000000000000000000, 0.000000000000000000, 1.000000000000000000 ) ) ;
#11164=CYLINDRICAL_SURFACE ( 'NONE', #12552, 25.00000000000000000 ) ;
#11233=EDGE_CURVE ( 'NONE', #2030, #2015, #5272, .T. ) ;
#11235=CARTESIAN_POINT ( 'NONE',  ( 13.00000000000000178, 20.00000000000000000, -11.32475165290605901 ) ) ;
#11243=UNCERTAINTY_MEASURE_WITH_UNIT (LENGTH_MEASURE( 1.000000000000000082E-05 ), #17257, 'distance_accuracy_value', 'NONE');
#11244=VECTOR ( 'NONE', #6041, 1000.000000000000000 ) ;
#11266=AXIS2_PLACEMENT_3D ( 'NONE', #17167, #4921, #1589 ) ;
#11275=VERTEX_POINT ( 'NONE', #13844 ) ;
#11326=CARTESIAN_POINT ( 'NONE',  ( -6.000000000000000000, -20.00000000000000000, -5.999999999999999112 ) ) ;
#11331=CIRCLE ( 'NONE', #4017, 16.49999999999998579 ) ;
#11344=CARTESIAN_POINT ( 'NONE',  ( -6.000000000000000000, 20.00000000000000000, -5.999999999999999112 ) ) ;
#11347=DIRECTION ( 'NONE',  ( -0.000000000000000000, -1.000000000000000000, -0.000000000000000000 ) ) ;
#11352=EDGE_CURVE ( 'NONE', #407, #8973, #19708, .T. ) ;
#11356=DIRECTION ( 'NONE',  ( -3.063596499322173499E-16, 0.000000000000000000, 1.000000000000000000 ) ) ;
#11433=CARTESIAN_POINT ( 'NONE',  ( 1.734723475976807094E-14, 20.00000000000000000, 20.71067811865476216 ) ) ;
#11461=DIRECTION ( 'NONE',  ( -1.445602896647339410E-16, -0.000000000000000000, -1.000000000000000000 ) ) ;
#11466=CARTESIAN_POINT ( 'NONE',  ( -25.00000000000000000, -20.00000000000000000, -16.49999999999998934 ) ) ;
#11481=VERTEX_POINT ( 'NONE', #788 ) ;
#11526=CARTESIAN_POINT ( 'NONE',  ( -12.99999999999999467, -20.00000000000000000, 11.32475165290612296 ) ) ;
#11536=DIRECTION ( 'NONE',  ( 0.000000000000000000, 0.000000000000000000, -1.000000000000000000 ) ) ;
#11540=DIRECTION ( 'NONE',  ( 0.000000000000000000, 0.000000000000000000, -1.000000000000000000 ) ) ;
#11565=VERTEX_POINT ( 'NONE', #12311 ) ;
#11566=VECTOR ( 'NONE', #11461, 1000.000000000000000 ) ;
#11582=DIRECTION ( 'NONE',  ( -0.000000000000000000, -1.000000000000000000, 0.000000000000000000 ) ) ;
#11600=LINE ( 'NONE', #18595, #22603 ) ;
#11671=EDGE_CURVE ( 'NONE', #20094, #14167, #3765, .T. ) ;
#11696=ORIENTED_EDGE ( 'NONE', *, *, #14205, .F. ) ;
#11702=DIRECTION ( 'NONE',  ( -0.000000000000000000, -1.000000000000000000, -0.000000000000000000 ) ) ;
#11709=ORIENTED_EDGE ( 'NONE', *, *, #9920, .F. ) ;
#11767=VERTEX_POINT ( 'NONE', #18265 ) ;
#11785=ORIENTED_EDGE ( 'NONE', *, *, #476, .F. ) ;
#11789=CARTESIAN_POINT ( 'NONE',  ( 5.999999999999998224, 20.00000000000000000, -5.999999999999999112 ) ) ;
#11793=CARTESIAN_POINT ( 'NONE',  ( -25.00000000000000000, 20.00000000000000000, 6.487780019669002523E-15 ) ) ;
#11807=DIRECTION ( 'NONE',  ( -0.000000000000000000, -1.000000000000000000, -0.000000000000000000 ) ) ;
#11896=CIRCLE ( 'NONE', #21421, 25.00000000000000711 ) ;
#11917=EDGE_CURVE ( 'NONE', #2015, #5630, #16654, .T. ) ;
#11926=ORIENTED_EDGE ( 'NONE', *, *, #15758, .F. ) ;
#11943=VECTOR ( 'NONE', #21300, 1000.000000000000000 ) ;
#12023=FACE_OUTER_BOUND ( 'NONE', #8233, .T. ) ;
#12042=VERTEX_POINT ( 'NONE', #13877 ) ;
#12045=CIRCLE ( 'NONE', #14593, 25.00000000000000000 ) ;
#12091=DIRECTION ( 'NONE',  ( -0.000000000000000000, -1.000000000000000000, -0.000000000000000000 ) ) ;
#12104=CIRCLE ( 'NONE', #2229, 16.49999999999999645 ) ;
#12230=APPLICATION_CONTEXT ( 'automotive_design' ) ;
#12266=ORIENTED_EDGE ( 'NONE', *, *, #1382, .T. ) ;
#12295=EDGE_CURVE ( 'NONE', #1418, #7291, #16953, .T. ) ;
#12311=CARTESIAN_POINT ( 'NONE',  ( -25.00000000000000000, -20.00000000000000000, -25.00000000000000000 ) ) ;
#12340=AXIS2_PLACEMENT_3D ( 'NONE', #6903, #1741, #18930 ) ;
#12397=ORIENTED_EDGE ( 'NONE', *, *, #14634, .F. ) ;
#12436=( NAMED_UNIT ( * ) SI_UNIT ( $, .STERADIAN. ) SOLID_ANGLE_UNIT ( ) );
#12461=AXIS2_PLACEMENT_3D ( 'NONE', #19965, #4276, #9761 ) ;
#12481=EDGE_LOOP ( 'NONE', ( #16641, #15937, #19423, #21834 ) ) ;
#12483=DIRECTION ( 'NONE',  ( 0.000000000000000000, 1.000000000000000000, 0.000000000000000000 ) ) ;
#12491=EDGE_CURVE ( 'NONE', #15447, #16688, #21363, .T. ) ;
#12537=VECTOR ( 'NONE', #19727, 1000.000000000000000 ) ;
#12552=AXIS2_PLACEMENT_3D ( 'NONE', #14363, #631, #10819 ) ;
#12553=ORIENTED_EDGE ( 'NONE', *, *, #17946, .T. ) ;
#12586=LINE ( 'NONE', #3910, #12537 ) ;
#12603=ADVANCED_FACE ( 'NONE', ( #4121 ), #10863, .T. ) ;
#12612=AXIS2_PLACEMENT_3D ( 'NONE', #22180, #2818, #13323 ) ;
#12617=DIRECTION ( 'NONE',  ( -0.000000000000000000, -1.000000000000000000, -0.000000000000000000 ) ) ;
#12624=ORIENTED_EDGE ( 'NONE', *, *, #190, .T. ) ;
#12643=ORIENTED_EDGE ( 'NONE', *, *, #9082, .T. ) ;
#12696=EDGE_LOOP ( 'NONE', ( #22417, #12784, #8369, #12397 ) ) ;
#12784=ORIENTED_EDGE ( 'NONE', *, *, #21089, .T. ) ;
#12785=AXIS2_PLACEMENT_3D ( 'NONE', #17789, #2094, #21015 ) ;
#12791=DIRECTION ( 'NONE',  ( 0.000000000000000000, 0.000000000000000000, -1.000000000000000000 ) ) ;
#12820=ORIENTED_EDGE ( 'NONE', *, *, #11671, .F. ) ;
#12865=ORIENTED_EDGE ( 'NONE', *, *, #10725, .F. ) ;
#12891=VERTEX_POINT ( 'NONE', #2970 ) ;
#12974=CARTESIAN_POINT ( 'NONE',  ( -6.000000000000000000, 20.00000000000000000, -5.999999999999999112 ) ) ;
#12982=ORIENTED_EDGE ( 'NONE', *, *, #13850, .T. ) ;
#12995=DIRECTION ( 'NONE',  ( 0.000000000000000000, 1.000000000000000000, 0.000000000000000000 ) ) ;
#13015=CARTESIAN_POINT ( 'NONE',  ( -16.66666666666666785, 20.00000000000000000, -23.57022603955158502 ) ) ;
#13019=CARTESIAN_POINT ( 'NONE',  ( -25.00000000000000000, 20.00000000000000000, 6.487780019669002523E-15 ) ) ;
#13021=LINE ( 'NONE', #11326, #11943 ) ;
#13023=ORIENTED_EDGE ( 'NONE', *, *, #6746, .T. ) ;
#13115=AXIS2_PLACEMENT_3D ( 'NONE', #18651, #16815, #21317 ) ;
#13232=CYLINDRICAL_SURFACE ( 'NONE', #1790, 16.49999999999999645 ) ;
#13261=ORIENTED_EDGE ( 'NONE', *, *, #9213, .F. ) ;
#13262=LINE ( 'NONE', #13601, #15607 ) ;
#13289=CARTESIAN_POINT ( 'NONE',  ( 25.00000000000000000, 20.00000000000000000, -24.99999999999999289 ) ) ;
#13310=ADVANCED_FACE ( 'NONE', ( #14832 ), #989, .F. ) ;
#13323=DIRECTION ( 'NONE',  ( 0.000000000000000000, 0.000000000000000000, -1.000000000000000000 ) ) ;
#13333=ORIENTED_EDGE ( 'NONE', *, *, #11233, .F. ) ;
#13451=CIRCLE ( 'NONE', #20813, 25.00000000000000711 ) ;
#13476=DIRECTION ( 'NONE',  ( 0.000000000000000000, 1.000000000000000000, 0.000000000000000000 ) ) ;
#13477=CYLINDRICAL_SURFACE ( 'NONE', #3102, 50.00000000000000000 ) ;
#13539=EDGE_CURVE ( 'NONE', #131, #2473, #14131, .T. ) ;
#13562=DIRECTION ( 'NONE',  ( 0.000000000000000000, 0.000000000000000000, -1.000000000000000000 ) ) ;
#13566=ORIENTED_EDGE ( 'NONE', *, *, #2839, .F. ) ;
#13601=CARTESIAN_POINT ( 'NONE',  ( 25.00000000000000355, 20.00000000000000000, 25.00000000000000711 ) ) ;
#13645=EDGE_CURVE ( 'NONE', #5630, #159, #18933, .T. ) ;
#13674=CIRCLE ( 'NONE', #15146, 16.49999999999998579 ) ;
#13693=CIRCLE ( 'NONE', #8222, 50.00000000000000000 ) ;
#13694=ORIENTED_EDGE ( 'NONE', *, *, #17824, .F. ) ;
#13699=DIRECTION ( 'NONE',  ( -0.000000000000000000, -1.000000000000000000, 0.000000000000000000 ) ) ;
#13713=DIRECTION ( 'NONE',  ( -0.000000000000000000, -1.000000000000000000, -0.000000000000000000 ) ) ;
#13721=AXIS2_PLACEMENT_3D ( 'NONE', #16298, #9884, #18358 ) ;
#13733=EDGE_LOOP ( 'NONE', ( #4796, #22375, #13757, #9850 ) ) ;
#13757=ORIENTED_EDGE ( 'NONE', *, *, #15688, .T. ) ;
#13844=CARTESIAN_POINT ( 'NONE',  ( 13.00000000000000178, -20.00000000000000000, -11.32475165290605901 ) ) ;
#13850=EDGE_CURVE ( 'NONE', #16688, #2421, #6048, .T. ) ;
#13877=CARTESIAN_POINT ( 'NONE',  ( -24.99999999999999645, -20.00000000000000000, 25.00000000000001421 ) ) ;
#13888=CARTESIAN_POINT ( 'NONE',  ( 6.000000000000000000, 20.00000000000000000, 5.999999999999999112 ) ) ;
#13898=EDGE_LOOP ( 'NONE', ( #10430, #3564, #257, #15132, #7698, #21790, #21674, #7985, #17793 ) ) ;
#13944=PLANE ( 'NONE',  #5281 ) ;
#13992=EDGE_CURVE ( 'NONE', #11767, #2030, #19140, .T. ) ;
#14088=CIRCLE ( 'NONE', #7176, 16.49999999999999645 ) ;
#14131=CIRCLE ( 'NONE', #13721, 25.00000000000000000 ) ;
#14154=ORIENTED_EDGE ( 'NONE', *, *, #18615, .T. ) ;
#14167=VERTEX_POINT ( 'NONE', #14524 ) ;
#14198=ORIENTED_EDGE ( 'NONE', *, *, #5126, .T. ) ;
#14205=EDGE_CURVE ( 'NONE', #10374, #17205, #13693, .T. ) ;
#14220=ORIENTED_EDGE ( 'NONE', *, *, #18515, .T. ) ;
#14244=ADVANCED_FACE ( 'NONE', ( #15080 ), #13477, .F. ) ;
#14250=ADVANCED_BREP_SHAPE_REPRESENTATION ( '', ( #17752, #18273 ), #17150 ) ;
#14287=CARTESIAN_POINT ( 'NONE',  ( 25.00000000000000000, 20.00000000000000000, -16.49999999999997868 ) ) ;
#14301=CARTESIAN_POINT ( 'NONE',  ( 25.00000000000000355, 20.00000000000000000, 25.00000000000000711 ) ) ;
#14315=CARTESIAN_POINT ( 'NONE',  ( 1.734723475976807094E-14, 20.00000000000000000, 20.71067811865476216 ) ) ;
#14326=( NAMED_UNIT ( * ) PLANE_ANGLE_UNIT ( ) SI_UNIT ( $, .RADIAN. ) );
#14363=CARTESIAN_POINT ( 'NONE',  ( 25.00000000000000000, 20.00000000000000000, 6.487780019669002523E-15 ) ) ;
#14374=CARTESIAN_POINT ( 'NONE',  ( 6.000000000000000000, -20.00000000000000000, 5.999999999999998224 ) ) ;
#14390=CIRCLE ( 'NONE', #7872, 50.00000000000000000 ) ;
#14396=PRODUCT_DEFINITION_SHAPE ( 'NONE', 'NONE',  #306 ) ;
#14422=ORIENTED_EDGE ( 'NONE', *, *, #15688, .F. ) ;
#14434=PLANE ( 'NONE',  #10438 ) ;
#14469=EDGE_CURVE ( 'NONE', #11481, #8384, #19590, .T. ) ;
#14476=CIRCLE ( 'NONE', #15931, 50.00000000000000000 ) ;
#14504=ORIENTED_EDGE ( 'NONE', *, *, #7749, .F. ) ;
#14521=ORIENTED_EDGE ( 'NONE', *, *, #21365, .T. ) ;
#14524=CARTESIAN_POINT ( 'NONE',  ( 25.00000000000000355, -20.00000000000000000, 25.00000000000000711 ) ) ;
#14545=DIRECTION ( 'NONE',  ( 0.000000000000000000, 0.000000000000000000, -1.000000000000000000 ) ) ;
#14556=CARTESIAN_POINT ( 'NONE',  ( 5.999999999999998224, 20.00000000000000000, -5.999999999999999112 ) ) ;
#14563=ORIENTED_EDGE ( 'NONE', *, *, #13539, .F. ) ;
#14566=CARTESIAN_POINT ( 'NONE',  ( 5.999999999999998224, 20.00000000000000000, -5.999999999999999112 ) ) ;
#14593=AXIS2_PLACEMENT_3D ( 'NONE', #2248, #16213, #11059 ) ;
#14622=ADVANCED_FACE ( 'NONE', ( #1071 ), #3121, .T. ) ;
#14634=EDGE_CURVE ( 'NONE', #8988, #131, #6330, .T. ) ;
#14663=DIRECTION ( 'NONE',  ( -0.000000000000000000, -1.000000000000000000, -0.000000000000000000 ) ) ;
#14715=CARTESIAN_POINT ( 'NONE',  ( 25.00000000000000000, -20.00000000000000000, 6.487780019669002523E-15 ) ) ;
#14732=DIRECTION ( 'NONE',  ( 0.000000000000000000, 0.000000000000000000, 1.000000000000000000 ) ) ;
#14774=CARTESIAN_POINT ( 'NONE',  ( 1.734723475976807094E-14, -20.00000000000000000, 20.71067811865476216 ) ) ;
#14776=DIRECTION ( 'NONE',  ( 1.445602896647339410E-16, 0.000000000000000000, 1.000000000000000000 ) ) ;
#14832=FACE_OUTER_BOUND ( 'NONE', #17355, .T. ) ;
#14892=ORIENTED_EDGE ( 'NONE', *, *, #16106, .T. ) ;
#14928=ORIENTED_EDGE ( 'NONE', *, *, #6337, .T. ) ;
#14931=CARTESIAN_POINT ( 'NONE',  ( -24.99999999999999645, 20.00000000000000000, 25.00000000000001421 ) ) ;
#14932=ORIENTED_EDGE ( 'NONE', *, *, #20868, .T. ) ;
#14993=CARTESIAN_POINT ( 'NONE',  ( 5.999999999999998224, -20.00000000000000000, -5.999999999999999112 ) ) ;
#14999=DIRECTION ( 'NONE',  ( 0.000000000000000000, 0.000000000000000000, 1.000000000000000000 ) ) ;
#15035=ORIENTED_EDGE ( 'NONE', *, *, #21645, .T. ) ;
#15077=ORIENTED_EDGE ( 'NONE', *, *, #15968, .T. ) ;
#15080=FACE_OUTER_BOUND ( 'NONE', #22316, .T. ) ;
#15132=ORIENTED_EDGE ( 'NONE', *, *, #18548, .T. ) ;
#15146=AXIS2_PLACEMENT_3D ( 'NONE', #4039, #18104, #8943 ) ;
#15154=CARTESIAN_POINT ( 'NONE',  ( -13.00000000000000178, 20.00000000000000000, -11.32475165290611407 ) ) ;
#15357=FACE_OUTER_BOUND ( 'NONE', #10961, .T. ) ;
#15362=DIRECTION ( 'NONE',  ( -1.000000000000000000, 0.000000000000000000, -0.000000000000000000 ) ) ;
#15372=CARTESIAN_POINT ( 'NONE',  ( -25.00000000000000000, 20.00000000000000000, 6.487780019669002523E-15 ) ) ;
#15407=CYLINDRICAL_SURFACE ( 'NONE', #8344, 25.00000000000000711 ) ;
#15418=CARTESIAN_POINT ( 'NONE',  ( 1.734723475976807094E-14, 20.00000000000000000, 70.71067811865476926 ) ) ;
#15421=CARTESIAN_POINT ( 'NONE',  ( -25.00000000000000000, -20.00000000000000000, 6.487780019669002523E-15 ) ) ;
#15441=DIRECTION ( 'NONE',  ( 0.000000000000000000, -0.000000000000000000, 1.000000000000000000 ) ) ;
#15447=VERTEX_POINT ( 'NONE', #3046 ) ;
#15491=DIRECTION ( 'NONE',  ( 0.000000000000000000, 0.000000000000000000, 1.000000000000000000 ) ) ;
#15559=VECTOR ( 'NONE', #18307, 1000.000000000000000 ) ;
#15578=CARTESIAN_POINT ( 'NONE',  ( 25.00000000000000000, 20.00000000000000000, 6.487780019669002523E-15 ) ) ;
#15607=VECTOR ( 'NONE', #1369, 1000.000000000000000 ) ;
#15608=VERTEX_POINT ( 'NONE', #5653 ) ;
#15630=VERTEX_POINT ( 'NONE', #3835 ) ;
#15673=CYLINDRICAL_SURFACE ( 'NONE', #8698, 16.49999999999999645 ) ;
#15688=EDGE_CURVE ( 'NONE', #7803, #17903, #5999, .T. ) ;
#15741=DIRECTION ( 'NONE',  ( 0.000000000000000000, 1.000000000000000000, 0.000000000000000000 ) ) ;
#15758=EDGE_CURVE ( 'NONE', #9978, #20188, #3095, .T. ) ;
#15778=CARTESIAN_POINT ( 'NONE',  ( 16.66666666666666430, 20.00000000000000000, 23.57022603955159212 ) ) ;
#15877=EDGE_CURVE ( 'NONE', #7803, #2693, #3442, .T. ) ;
#15900=DIRECTION ( 'NONE',  ( 1.000000000000000000, 0.000000000000000000, 0.000000000000000000 ) ) ;
#15931=AXIS2_PLACEMENT_3D ( 'NONE', #4602, #11582, #6763 ) ;
#15937=ORIENTED_EDGE ( 'NONE', *, *, #1069, .F. ) ;
#15956=ORIENTED_EDGE ( 'NONE', *, *, #3763, .T. ) ;
#15968=EDGE_CURVE ( 'NONE', #20188, #159, #13021, .T. ) ;
#16080=ORIENTED_EDGE ( 'NONE', *, *, #7997, .F. ) ;
#16105=CARTESIAN_POINT ( 'NONE',  ( -25.00000000000000000, 20.00000000000000000, 6.487780019669002523E-15 ) ) ;
#16106=EDGE_CURVE ( 'NONE', #10374, #19286, #22655, .T. ) ;
#16116=CARTESIAN_POINT ( 'NONE',  ( 13.00000000000000178, -20.00000000000000000, -11.32475165290605901 ) ) ;
#16150=FACE_BOUND ( 'NONE', #18148, .T. ) ;
#16213=DIRECTION ( 'NONE',  ( 0.000000000000000000, 1.000000000000000000, 0.000000000000000000 ) ) ;
#16224=VECTOR ( 'NONE', #4012, 1000.000000000000000 ) ;
#16225=VECTOR ( 'NONE', #11356, 1000.000000000000000 ) ;
#16278=ADVANCED_FACE ( 'NONE', ( #6459 ), #8507, .F. ) ;
#16298=CARTESIAN_POINT ( 'NONE',  ( 25.00000000000000000, -20.00000000000000000, 6.487780019669002523E-15 ) ) ;
#16308=PLANE ( 'NONE',  #18942 ) ;
#16342=DIRECTION ( 'NONE',  ( 0.000000000000000000, 0.000000000000000000, -1.000000000000000000 ) ) ;
#16349=EDGE_CURVE ( 'NONE', #12891, #7324, #11896, .T. ) ;
#16369=ORIENTED_EDGE ( 'NONE', *, *, #7775, .F. ) ;
#16511=VECTOR ( 'NONE', #11702, 1000.000000000000000 ) ;
#16528=DIRECTION ( 'NONE',  ( 0.000000000000000000, 1.000000000000000000, 0.000000000000000000 ) ) ;
#16566=EDGE_CURVE ( 'NONE', #7291, #11481, #243, .T. ) ;
#16635=ADVANCED_FACE ( 'NONE', ( #19952 ), #14434, .T. ) ;
#16641=ORIENTED_EDGE ( 'NONE', *, *, #12295, .F. ) ;
#16654=LINE ( 'NONE', #4754, #21337 ) ;
#16687=VERTEX_POINT ( 'NONE', #11466 ) ;
#16688=VERTEX_POINT ( 'NONE', #18454 ) ;
#16752=EDGE_CURVE ( 'NONE', #5200, #16771, #14088, .T. ) ;
#16771=VERTEX_POINT ( 'NONE', #4932 ) ;
#16772=UNCERTAINTY_MEASURE_WITH_UNIT (LENGTH_MEASURE( 1.000000000000000082E-05 ), #7360, 'distance_accuracy_value', 'NONE');
#16782=EDGE_CURVE ( 'NONE', #19286, #20094, #14476, .T. ) ;
#16815=DIRECTION ( 'NONE',  ( -0.000000000000000000, -1.000000000000000000, -0.000000000000000000 ) ) ;
#16830=DIRECTION ( 'NONE',  ( 0.000000000000000000, 0.000000000000000000, -1.000000000000000000 ) ) ;
#16857=ORIENTED_EDGE ( 'NONE', *, *, #4516, .T. ) ;
#16871=DIRECTION ( 'NONE',  ( -0.000000000000000000, -1.000000000000000000, -0.000000000000000000 ) ) ;
#16884=DIRECTION ( 'NONE',  ( -1.000000000000000000, -0.000000000000000000, -0.000000000000000000 ) ) ;
#16921=CARTESIAN_POINT ( 'NONE',  ( 25.00000000000000000, 20.00000000000000000, 6.487780019669002523E-15 ) ) ;
#16927=FACE_OUTER_BOUND ( 'NONE', #10761, .T. ) ;
#16953=LINE ( 'NONE', #11235, #16225 ) ;
#16966=PLANE ( 'NONE',  #7601 ) ;
#16993=DIRECTION ( 'NONE',  ( 1.000000000000000000, 0.000000000000000000, 0.000000000000000000 ) ) ;
#17038=DIRECTION ( 'NONE',  ( 0.000000000000000000, 0.000000000000000000, -1.000000000000000000 ) ) ;
#17041=EDGE_CURVE ( 'NONE', #2693, #5200, #4983, .T. ) ;
#17110=AXIS2_PLACEMENT_3D ( 'NONE', #4835, #11807, #9762 ) ;
#17150=( GEOMETRIC_REPRESENTATION_CONTEXT ( 3 ) GLOBAL_UNCERTAINTY_ASSIGNED_CONTEXT ( ( #16772 ) ) GLOBAL_UNIT_ASSIGNED_CONTEXT ( ( #7360, #14326, #5755 ) ) REPRESENTATION_CONTEXT ( 'NONE', 'WORKASPACE' ) );
#17167=CARTESIAN_POINT ( 'NONE',  ( -13.00000000000000178, 20.00000000000000000, -11.32475165290611407 ) ) ;
#17186=CIRCLE ( 'NONE', #12785, 16.49999999999998579 ) ;
#17203=ORIENTED_EDGE ( 'NONE', *, *, #17041, .T. ) ;
#17205=VERTEX_POINT ( 'NONE', #22034 ) ;
#17232=CARTESIAN_POINT ( 'NONE',  ( -13.00000000000000000, -20.00000000000000000, -11.32475165290611230 ) ) ;
#17257=( LENGTH_UNIT ( ) NAMED_UNIT ( * ) SI_UNIT ( .MILLI., .METRE. ) );
#17339=ORIENTED_EDGE ( 'NONE', *, *, #1382, .F. ) ;
#17355=EDGE_LOOP ( 'NONE', ( #19553, #14154, #8522, #5715 ) ) ;
#17401=DIRECTION ( 'NONE',  ( -1.445602896647339410E-16, -0.000000000000000000, -1.000000000000000000 ) ) ;
#17410=ORIENTED_EDGE ( 'NONE', *, *, #3860, .T. ) ;
#17471=ORIENTED_EDGE ( 'NONE', *, *, #190, .F. ) ;
#17521=FACE_OUTER_BOUND ( 'NONE', #2095, .T. ) ;
#17575=AXIS2_PLACEMENT_3D ( 'NONE', #602, #723, #18247 ) ;
#17595=CARTESIAN_POINT ( 'NONE',  ( 16.66666666666669272, -20.00000000000000000, -23.57022603955159212 ) ) ;
#17671=EDGE_CURVE ( 'NONE', #8384, #8973, #10774, .T. ) ;
#17752=MANIFOLD_SOLID_BREP ( 'Boss-Extrude1', #3484 ) ;
#17762=VERTEX_POINT ( 'NONE', #1911 ) ;
#17783=EDGE_CURVE ( 'NONE', #14167, #131, #3283, .T. ) ;
#17787=APPLICATION_CONTEXT ( 'automotive_design' ) ;
#17789=CARTESIAN_POINT ( 'NONE',  ( 25.00000000000000000, 20.00000000000000000, 6.487780019669002523E-15 ) ) ;
#17793=ORIENTED_EDGE ( 'NONE', *, *, #17824, .T. ) ;
#17809=AXIS2_PLACEMENT_3D ( 'NONE', #18054, #9360, #16342 ) ;
#17824=EDGE_CURVE ( 'NONE', #8988, #15447, #12045, .T. ) ;
#17903=VERTEX_POINT ( 'NONE', #11526 ) ;
#17908=EDGE_LOOP ( 'NONE', ( #4269, #14932, #17471, #9437 ) ) ;
#17911=ORIENTED_EDGE ( 'NONE', *, *, #18661, .T. ) ;
#17912=CARTESIAN_POINT ( 'NONE',  ( 25.00000000000000000, 20.00000000000000000, -24.99999999999999289 ) ) ;
#17945=FACE_OUTER_BOUND ( 'NONE', #20155, .T. ) ;
#17946=EDGE_CURVE ( 'NONE', #7291, #15608, #11331, .T. ) ;
#17989=DIRECTION ( 'NONE',  ( -0.000000000000000000, -1.000000000000000000, -0.000000000000000000 ) ) ;
#17995=PLANE ( 'NONE',  #1413 ) ;
#18054=CARTESIAN_POINT ( 'NONE',  ( 25.00000000000000000, 20.00000000000000000, 6.487780019669002523E-15 ) ) ;
#18087=ORIENTED_EDGE ( 'NONE', *, *, #6028, .T. ) ;
#18104=DIRECTION ( 'NONE',  ( 0.000000000000000000, 1.000000000000000000, -0.000000000000000000 ) ) ;
#18124=ORIENTED_EDGE ( 'NONE', *, *, #15877, .F. ) ;
#18148=EDGE_LOOP ( 'NONE', ( #18263, #13333, #8594, #3585 ) ) ;
#18165=FACE_OUTER_BOUND ( 'NONE', #12696, .T. ) ;
#18207=VECTOR ( 'NONE', #20392, 1000.000000000000000 ) ;
#18236=AXIS2_PLACEMENT_3D ( 'NONE', #1909, #3749, #2019 ) ;
#18247=DIRECTION ( 'NONE',  ( 0.000000000000000000, 0.000000000000000000, -1.000000000000000000 ) ) ;
#18251=CARTESIAN_POINT ( 'NONE',  ( -5.999999999999998224, 20.00000000000000000, 5.999999999999999112 ) ) ;
#18263=ORIENTED_EDGE ( 'NONE', *, *, #11917, .F. ) ;
#18265=CARTESIAN_POINT ( 'NONE',  ( -5.999999999999996447, 20.00000000000000000, 5.999999999999998224 ) ) ;
#18273=AXIS2_PLACEMENT_3D ( 'NONE', #1648, #15491, #16993 ) ;
#18289=ADVANCED_FACE ( 'NONE', ( #16927 ), #9835, .F. ) ;
#18295=AXIS2_PLACEMENT_3D ( 'NONE', #16105, #6030, #2250 ) ;
#18307=DIRECTION ( 'NONE',  ( -0.000000000000000000, -1.000000000000000000, -0.000000000000000000 ) ) ;
#18358=DIRECTION ( 'NONE',  ( 0.000000000000000000, 0.000000000000000000, 1.000000000000000000 ) ) ;
#18362=ORIENTED_EDGE ( 'NONE', *, *, #21365, .F. ) ;
#18404=CARTESIAN_POINT ( 'NONE',  ( -6.000000000000000000, 20.00000000000000000, -5.999999999999999112 ) ) ;
#18423=DIRECTION ( 'NONE',  ( -0.000000000000000000, -1.000000000000000000, -0.000000000000000000 ) ) ;
#18454=CARTESIAN_POINT ( 'NONE',  ( -16.66666666666666785, 20.00000000000000000, -23.57022603955158502 ) ) ;
#18458=ORIENTED_EDGE ( 'NONE', *, *, #21645, .F. ) ;
#18464=CARTESIAN_POINT ( 'NONE',  ( -6.000000000000000000, 20.00000000000000000, -5.999999999999999112 ) ) ;
#18515=EDGE_CURVE ( 'NONE', #7324, #12042, #19790, .T. ) ;
#18536=ADVANCED_FACE ( 'NONE', ( #17945 ), #7405, .F. ) ;
#18548=EDGE_CURVE ( 'NONE', #7324, #17762, #2198, .T. ) ;
#18595=CARTESIAN_POINT ( 'NONE',  ( 13.00000000000000178, 20.00000000000000000, -11.32475165290605901 ) ) ;
#18615=EDGE_CURVE ( 'NONE', #15608, #407, #17186, .T. ) ;
#18637=AXIS2_PLACEMENT_3D ( 'NONE', #14715, #12995, #21502 ) ;
#18641=PRODUCT_DEFINITION_FORMATION_WITH_SPECIFIED_SOURCE ( 'ANY', '', #5829, .NOT_KNOWN. ) ;
#18651=CARTESIAN_POINT ( 'NONE',  ( 25.00000000000000000, 20.00000000000000000, 6.487780019669002523E-15 ) ) ;
#18661=EDGE_CURVE ( 'NONE', #8973, #11275, #19780, .T. ) ;
#18773=AXIS2_PLACEMENT_3D ( 'NONE', #8772, #15741, #53 ) ;
#18836=AXIS2_PLACEMENT_3D ( 'NONE', #15421, #13476, #18884 ) ;
#18849=EDGE_LOOP ( 'NONE', ( #13261, #1820, #21469, #14198 ) ) ;
#18858=ADVANCED_FACE ( 'NONE', ( #6555 ), #16966, .T. ) ;
#18863=ADVANCED_FACE ( 'NONE', ( #20532 ), #8382, .F. ) ;
#18884=DIRECTION ( 'NONE',  ( 0.000000000000000000, 0.000000000000000000, 1.000000000000000000 ) ) ;
#18908=FACE_BOUND ( 'NONE', #7549, .T. ) ;
#18930=DIRECTION ( 'NONE',  ( 0.000000000000000000, 0.000000000000000000, 1.000000000000000000 ) ) ;
#18933=LINE ( 'NONE', #20542, #8623 ) ;
#18942=AXIS2_PLACEMENT_3D ( 'NONE', #12974, #7608, #5892 ) ;
#18946=EDGE_CURVE ( 'NONE', #8364, #8988, #6866, .T. ) ;
#18951=ORIENTED_EDGE ( 'NONE', *, *, #7775, .T. ) ;
#19070=ADVANCED_FACE ( 'NONE', ( #21704 ), #16308, .T. ) ;
#19085=ADVANCED_FACE ( 'NONE', ( #6458 ), #10217, .T. ) ;
#19105=CIRCLE ( 'NONE', #814, 50.00000000000001421 ) ;
#19109=ORIENTED_EDGE ( 'NONE', *, *, #9213, .T. ) ;
#19140=LINE ( 'NONE', #5492, #3521 ) ;
#19204=AXIS2_PLACEMENT_3D ( 'NONE', #9774, #20544, #3124 ) ;
#19286=VERTEX_POINT ( 'NONE', #14774 ) ;
#19298=DIRECTION ( 'NONE',  ( -0.000000000000000000, -1.000000000000000000, -0.000000000000000000 ) ) ;
#19357=VECTOR ( 'NONE', #5128, 1000.000000000000000 ) ;
#19358=VECTOR ( 'NONE', #2913, 1000.000000000000000 ) ;
#19423=ORIENTED_EDGE ( 'NONE', *, *, #18615, .F. ) ;
#19440=CARTESIAN_POINT ( 'NONE',  ( -13.00000000000000178, -20.00000000000000000, -11.32475165290611407 ) ) ;
#19544=ORIENTED_EDGE ( 'NONE', *, *, #3763, .F. ) ;
#19553=ORIENTED_EDGE ( 'NONE', *, *, #21083, .F. ) ;
#19590=CIRCLE ( 'NONE', #12612, 16.49999999999998579 ) ;
#19602=ORIENTED_EDGE ( 'NONE', *, *, #17783, .F. ) ;
#19603=FACE_OUTER_BOUND ( 'NONE', #13733, .T. ) ;
#19651=LINE ( 'NONE', #11038, #2468 ) ;
#19670=CARTESIAN_POINT ( 'NONE',  ( 16.66666666666666430, -20.00000000000000000, 23.57022603955159212 ) ) ;
#19685=ADVANCED_FACE ( 'NONE', ( #2728 ), #455, .T. ) ;
#19700=AXIS2_PLACEMENT_3D ( 'NONE', #4980, #22405, #1773 ) ;
#19708=LINE ( 'NONE', #14287, #16224 ) ;
#19727=DIRECTION ( 'NONE',  ( -0.000000000000000000, -1.000000000000000000, -0.000000000000000000 ) ) ;
#19734=ADVANCED_FACE ( 'NONE', ( #8000 ), #20255, .F. ) ;
#19754=CARTESIAN_POINT ( 'NONE',  ( -24.99999999999999645, -20.00000000000000000, 16.50000000000000355 ) ) ;
#19755=LINE ( 'NONE', #18251, #3955 ) ;
#19780=CIRCLE ( 'NONE', #17575, 16.49999999999998579 ) ;
#19790=LINE ( 'NONE', #3864, #3668 ) ;
#19793=ADVANCED_FACE ( 'NONE', ( #19603 ), #13232, .F. ) ;
#19825=ORIENTED_EDGE ( 'NONE', *, *, #16566, .T. ) ;
#19927=CIRCLE ( 'NONE', #19204, 25.00000000000000711 ) ;
#19944=ORIENTED_EDGE ( 'NONE', *, *, #11917, .T. ) ;
#19952=FACE_OUTER_BOUND ( 'NONE', #20923, .T. ) ;
#19965=CARTESIAN_POINT ( 'NONE',  ( 1.734723475976807094E-14, 20.00000000000000000, 70.71067811865476926 ) ) ;
#19988=ORIENTED_EDGE ( 'NONE', *, *, #16752, .F. ) ;
#20094=VERTEX_POINT ( 'NONE', #19670 ) ;
#20128=DIRECTION ( 'NONE',  ( 0.000000000000000000, 0.000000000000000000, -1.000000000000000000 ) ) ;
#20155=EDGE_LOOP ( 'NONE', ( #4517, #7412, #12643, #7671 ) ) ;
#20188=VERTEX_POINT ( 'NONE', #4657 ) ;
#20252=CARTESIAN_POINT ( 'NONE',  ( -25.00000000000000000, 20.00000000000000000, 6.487780019669002523E-15 ) ) ;
#20255=CYLINDRICAL_SURFACE ( 'NONE', #21177, 16.49999999999998579 ) ;
#20289=CARTESIAN_POINT ( 'NONE',  ( 1.734723475976807094E-14, -20.00000000000000000, -70.71067811865476926 ) ) ;
#20306=ORIENTED_EDGE ( 'NONE', *, *, #16782, .T. ) ;
#20346=VECTOR ( 'NONE', #5516, 1000.000000000000000 ) ;
#20392=DIRECTION ( 'NONE',  ( -0.000000000000000000, -1.000000000000000000, -0.000000000000000000 ) ) ;
#20404=CIRCLE ( 'NONE', #12340, 16.49999999999999645 ) ;
#20439=DIRECTION ( 'NONE',  ( 0.000000000000000000, 0.000000000000000000, -1.000000000000000000 ) ) ;
#20446=DIRECTION ( 'NONE',  ( -0.000000000000000000, -1.000000000000000000, -0.000000000000000000 ) ) ;
#20493=CARTESIAN_POINT ( 'NONE',  ( 1.734723475976807094E-14, 20.00000000000000000, 70.71067811865476926 ) ) ;
#20532=FACE_OUTER_BOUND ( 'NONE', #17908, .T. ) ;
#20542=CARTESIAN_POINT ( 'NONE',  ( -6.000000000000000000, 20.00000000000000000, -5.999999999999999112 ) ) ;
#20544=DIRECTION ( 'NONE',  ( 0.000000000000000000, 1.000000000000000000, 0.000000000000000000 ) ) ;
#20585=VECTOR ( 'NONE', #13713, 1000.000000000000000 ) ;
#20666=ADVANCED_FACE ( 'NONE', ( #8396 ), #6675, .T. ) ;
#20729=AXIS2_PLACEMENT_3D ( 'NONE', #4958, #9987, #20439 ) ;
#20813=AXIS2_PLACEMENT_3D ( 'NONE', #779, #4449, #14732 ) ;
#20868=EDGE_CURVE ( 'NONE', #16771, #2945, #1858, .T. ) ;
#20894=CARTESIAN_POINT ( 'NONE',  ( 12.99999999999999467, 20.00000000000000000, 11.32475165290614960 ) ) ;
#20923=EDGE_LOOP ( 'NONE', ( #11926, #16369, #9989, #568 ) ) ;
#20985=VERTEX_POINT ( 'NONE', #704 ) ;
#21015=DIRECTION ( 'NONE',  ( 0.000000000000000000, 0.000000000000000000, -1.000000000000000000 ) ) ;
#21081=DIRECTION ( 'NONE',  ( 3.063596499322173499E-16, 0.000000000000000000, -1.000000000000000000 ) ) ;
#21083=EDGE_CURVE ( 'NONE', #15608, #8384, #1146, .T. ) ;
#21089=EDGE_CURVE ( 'NONE', #8364, #14167, #13262, .T. ) ;
#21166=CIRCLE ( 'NONE', #19700, 25.00000000000000711 ) ;
#21177=AXIS2_PLACEMENT_3D ( 'NONE', #16921, #5613, #14545 ) ;
#21271=PRODUCT_DEFINITION_CONTEXT ( 'detailed design', #17787, 'design' ) ;
#21300=DIRECTION ( 'NONE',  ( -1.000000000000000000, -0.000000000000000000, -0.000000000000000000 ) ) ;
#21317=DIRECTION ( 'NONE',  ( 0.000000000000000000, 0.000000000000000000, -1.000000000000000000 ) ) ;
#21337=VECTOR ( 'NONE', #16884, 1000.000000000000000 ) ;
#21363=CIRCLE ( 'NONE', #10721, 50.00000000000001421 ) ;
#21365=EDGE_CURVE ( 'NONE', #15447, #2473, #19651, .T. ) ;
#21388=DIRECTION ( 'NONE',  ( -0.000000000000000000, -1.000000000000000000, -0.000000000000000000 ) ) ;
#21421=AXIS2_PLACEMENT_3D ( 'NONE', #5089, #8175, #10219 ) ;
#21469=ORIENTED_EDGE ( 'NONE', *, *, #21827, .T. ) ;
#21502=DIRECTION ( 'NONE',  ( 0.000000000000000000, 0.000000000000000000, 1.000000000000000000 ) ) ;
#21521=DIRECTION ( 'NONE',  ( -0.000000000000000000, -1.000000000000000000, -0.000000000000000000 ) ) ;
#21522=DIRECTION ( 'NONE',  ( -0.000000000000000000, -1.000000000000000000, -0.000000000000000000 ) ) ;
#21561=FACE_BOUND ( 'NONE', #12481, .T. ) ;
#21573=EDGE_LOOP ( 'NONE', ( #12553, #3261, #3856, #10409 ) ) ;
#21576=CARTESIAN_POINT ( 'NONE',  ( 6.000000000000000000, 20.00000000000000000, 5.999999999999999112 ) ) ;
#21638=DIRECTION ( 'NONE',  ( 0.000000000000000000, 0.000000000000000000, 1.000000000000000000 ) ) ;
#21645=EDGE_CURVE ( 'NONE', #12891, #11565, #5034, .T. ) ;
#21674=ORIENTED_EDGE ( 'NONE', *, *, #10725, .T. ) ;
#21704=FACE_OUTER_BOUND ( 'NONE', #2174, .T. ) ;
#21724=VECTOR ( 'NONE', #17401, 1000.000000000000000 ) ;
#21790=ORIENTED_EDGE ( 'NONE', *, *, #14205, .T. ) ;
#21827=EDGE_CURVE ( 'NONE', #5630, #11767, #2378, .T. ) ;
#21834=ORIENTED_EDGE ( 'NONE', *, *, #17946, .F. ) ;
#21901=DIRECTION ( 'NONE',  ( 0.000000000000000000, 0.000000000000000000, 1.000000000000000000 ) ) ;
#21947=ADVANCED_FACE ( 'NONE', ( #8105 ), #15407, .T. ) ;
#22009=CARTESIAN_POINT ( 'NONE',  ( 25.00000000000000355, 20.00000000000000000, 16.49999999999999289 ) ) ;
#22034=CARTESIAN_POINT ( 'NONE',  ( 16.66666666666666430, 20.00000000000000000, 23.57022603955159212 ) ) ;
#22138=LINE ( 'NONE', #6436, #16511 ) ;
#22168=ORIENTED_EDGE ( 'NONE', *, *, #13850, .F. ) ;
#22180=CARTESIAN_POINT ( 'NONE',  ( 25.00000000000000000, -20.00000000000000000, 6.487780019669002523E-15 ) ) ;
#22316=EDGE_LOOP ( 'NONE', ( #9368, #16080, #14928, #7938 ) ) ;
#22353=DIRECTION ( 'NONE',  ( -0.000000000000000000, -1.000000000000000000, -0.000000000000000000 ) ) ;
#22371=CIRCLE ( 'NONE', #12461, 50.00000000000000000 ) ;
#22375=ORIENTED_EDGE ( 'NONE', *, *, #7749, .T. ) ;
#22405=DIRECTION ( 'NONE',  ( 0.000000000000000000, 1.000000000000000000, 0.000000000000000000 ) ) ;
#22417=ORIENTED_EDGE ( 'NONE', *, *, #18946, .F. ) ;
#22488=ORIENTED_EDGE ( 'NONE', *, *, #893, .F. ) ;
#22490=CARTESIAN_POINT ( 'NONE',  ( -6.000000000000000000, -20.00000000000000000, -5.999999999999999112 ) ) ;
#22495=ORIENTED_EDGE ( 'NONE', *, *, #6337, .F. ) ;
#22601=DIRECTION ( 'NONE',  ( 0.000000000000000000, 0.000000000000000000, 1.000000000000000000 ) ) ;
#22603=VECTOR ( 'NONE', #16871, 1000.000000000000000 ) ;
#22655=LINE ( 'NONE', #11433, #4227 ) ;
#22666=ORIENTED_EDGE ( 'NONE', *, *, #6028, .F. ) ;
#22714=COLOUR_RGB('Light Blue',0.38,0.62,0.78);
#22715=FILL_AREA_STYLE_COLOUR('',#22714);
#22716=FILL_AREA_STYLE('',(#22715));
#22717=SURFACE_STYLE_FILL_AREA(#22716);
#22718=SURFACE_SIDE_STYLE('',(#22717));
#22719=SURFACE_STYLE_USAGE(.BOTH.,#22718);
#22720=PRESENTATION_STYLE_ASSIGNMENT((#22719));
ENDSEC;
END-ISO-10303-21;
